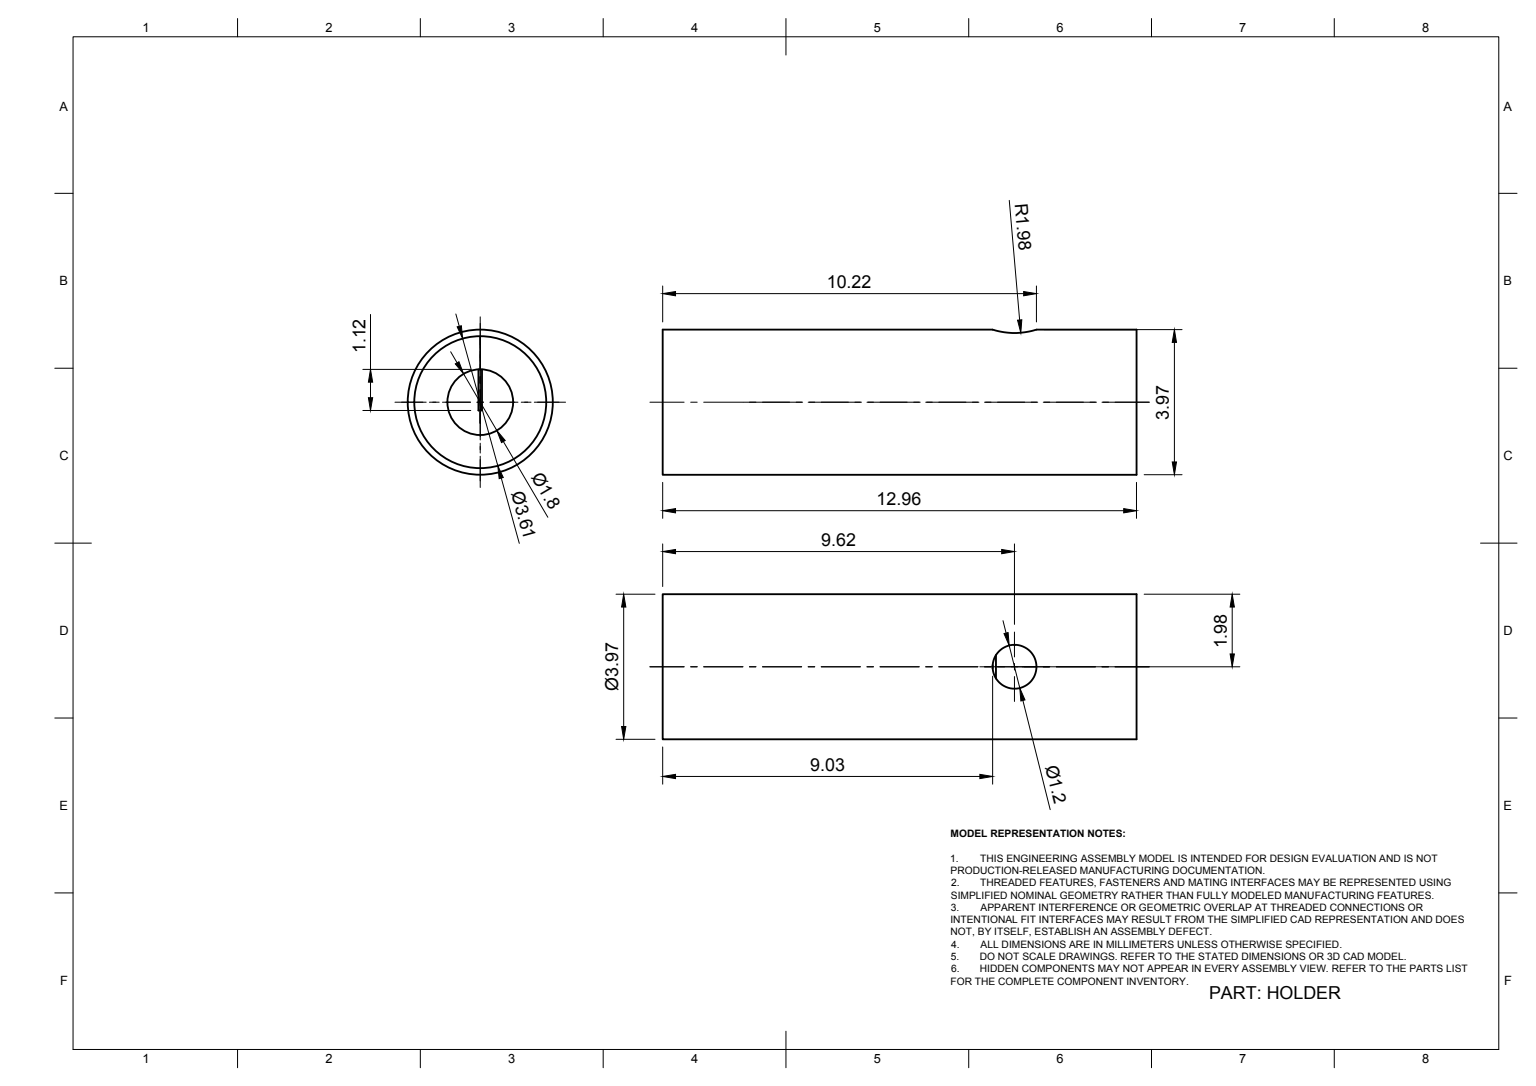
ISO-10303-21;
HEADER;
/* Generated by software containing ST-Developer
 * from STEP Tools, Inc. (www.steptools.com) 
 */

FILE_DESCRIPTION(
/* description */ (''),
/* implementation_level */ '2;1');

FILE_NAME(
/* name */ 'Holder.step',
/* time_stamp */ '2026-10-05T00:51:14-07:00',
/* author */ (''),
/* organization */ (''),
/* preprocessor_version */ 'ST-DEVELOPER v20.2',
/* originating_system */ 'Autodesk Translation Framework v15.15.0.0',
/* authorisation */ '');

FILE_SCHEMA (('AUTOMOTIVE_DESIGN { 1 0 10303 214 3 1 1 }'));
ENDSEC;

DATA;
#10=MECHANICAL_DESIGN_GEOMETRIC_PRESENTATION_REPRESENTATION('',(#388),#4613);
#48=CONICAL_SURFACE('',#1711,1.35128847266969,0.789744339373133);
#67=FACE_BOUND('',#517,.T.);
#68=FACE_BOUND('',#522,.T.);
#69=FACE_BOUND('',#525,.T.);
#70=FACE_BOUND('',#528,.T.);
#91=PLANE('',#1698);
#92=PLANE('',#1702);
#93=PLANE('',#1706);
#94=PLANE('',#1707);
#95=PLANE('',#1715);
#96=PLANE('',#1719);
#97=PLANE('',#1723);
#98=PLANE('',#1727);
#132=B_SPLINE_CURVE_WITH_KNOTS('',3,(#2423,#2424,#2425,#2426,#2427,#2428),
 .UNSPECIFIED.,.F.,.F.,(4,2,4),(0.0611341523507192,0.0707646671678304,0.089396591469994),
 .UNSPECIFIED.);
#133=B_SPLINE_CURVE_WITH_KNOTS('',3,(#2432,#2433,#2434,#2435,#2436,#2437,
#2438,#2439,#2440,#2441,#2442,#2443,#2444,#2445,#2446,#2447,#2448),
 .UNSPECIFIED.,.F.,.F.,(4,2,2,2,3,2,2,4),(-0.0922607888499982,-0.0692273118115021,
-0.0461938347730059,-0.023096917386503,0.,0.023096917386503,0.0461938347730059,
0.0596041129805193),.UNSPECIFIED.);
#134=B_SPLINE_CURVE_WITH_KNOTS('',3,(#2452,#2453,#2454,#2455,#2456,#2457,
#2458,#2459,#2460,#2461),.UNSPECIFIED.,.F.,.F.,(4,2,2,2,4),(0.,0.0227593204764388,
0.0455186409528775,0.0682709506447675,0.0910232603366575),.UNSPECIFIED.);
#135=B_SPLINE_CURVE_WITH_KNOTS('',3,(#2463,#2464,#2465,#2466,#2467,#2468,
#2469,#2470,#2471,#2472),.UNSPECIFIED.,.F.,.F.,(4,2,2,2,4),(0.273069781009973,
0.295822090701863,0.318574400393753,0.341333720870191,0.36409304134663),
 .UNSPECIFIED.);
#136=B_SPLINE_CURVE_WITH_KNOTS('',3,(#2473,#2474,#2475,#2476,#2477,#2478,
#2479,#2480,#2481,#2482,#2483,#2484,#2485,#2486,#2487,#2488,#2489,#2490),
 .UNSPECIFIED.,.F.,.F.,(4,2,2,2,2,2,2,2,4),(0.0910232603366575,0.113775570028548,
0.136527879720438,0.159287200196876,0.182046520673315,0.204805841149754,
0.227565161626193,0.250317471318083,0.273069781009973),.UNSPECIFIED.);
#137=B_SPLINE_CURVE_WITH_KNOTS('',3,(#2492,#2493,#2494,#2495,#2496,#2497,
#2498,#2499,#2500,#2501,#2502,#2503,#2504,#2505,#2506,#2507),
 .UNSPECIFIED.,.F.,.F.,(4,2,2,2,2,2,2,4),(-0.244125690634136,-0.230715412473002,
-0.207618495086499,-0.184521577699996,-0.161424660313493,-0.13832774292699,
-0.115294265888494,-0.0922607888499982),.UNSPECIFIED.);
#138=B_SPLINE_CURVE_WITH_KNOTS('',3,(#2510,#2511,#2512,#2513,#2514,#2515),
 .UNSPECIFIED.,.F.,.F.,(4,2,4),(0.0989596757247573,0.117591600026921,0.127222114844032),
 .UNSPECIFIED.);
#165=LINE('',#2417,#248);
#166=LINE('',#2421,#249);
#167=LINE('',#2430,#250);
#168=LINE('',#2450,#251);
#169=LINE('',#2509,#252);
#170=LINE('',#2517,#253);
#171=LINE('',#2521,#254);
#172=LINE('',#2534,#255);
#173=LINE('',#2537,#256);
#174=LINE('',#2542,#257);
#175=LINE('',#2549,#258);
#176=LINE('',#2550,#259);
#177=LINE('',#2557,#260);
#178=LINE('',#2564,#261);
#248=VECTOR('',#1914,10.);
#249=VECTOR('',#1917,10.);
#250=VECTOR('',#1918,10.);
#251=VECTOR('',#1919,0.600000000000001);
#252=VECTOR('',#1920,10.);
#253=VECTOR('',#1923,10.);
#254=VECTOR('',#1928,1.19802042656629);
#255=VECTOR('',#1949,0.898903149093028);
#256=VECTOR('',#1952,1.35128847266969);
#257=VECTOR('',#1959,1.80367379624636);
#258=VECTOR('',#1968,1.9840612380693);
#259=VECTOR('',#1969,1.9840612380693);
#260=VECTOR('',#1978,1.49577760563294);
#261=VECTOR('',#1987,1.24385197034191);
#331=CYLINDRICAL_SURFACE('',#1696,0.600000000000001);
#332=CYLINDRICAL_SURFACE('',#1699,1.19802042656629);
#333=CYLINDRICAL_SURFACE('',#1704,0.898903149093028);
#334=CYLINDRICAL_SURFACE('',#1709,0.898903149093028);
#335=CYLINDRICAL_SURFACE('',#1713,1.80367379624636);
#336=CYLINDRICAL_SURFACE('',#1717,1.9840612380693);
#337=CYLINDRICAL_SURFACE('',#1721,1.49577760563294);
#338=CYLINDRICAL_SURFACE('',#1725,1.24385197034191);
#372=SHAPE_REPRESENTATION_RELATIONSHIP('SRR','None',#4646,#380);
#380=ADVANCED_BREP_SHAPE_REPRESENTATION('',(#396),#4606);
#388=STYLED_ITEM('',(#4695),#396);
#396=MANIFOLD_SOLID_BREP('Body1',#1595);
#404=FACE_OUTER_BOUND('',#510,.T.);
#405=FACE_OUTER_BOUND('',#511,.T.);
#406=FACE_OUTER_BOUND('',#512,.T.);
#407=FACE_OUTER_BOUND('',#513,.T.);
#408=FACE_OUTER_BOUND('',#514,.T.);
#409=FACE_OUTER_BOUND('',#515,.T.);
#410=FACE_OUTER_BOUND('',#516,.T.);
#411=FACE_OUTER_BOUND('',#518,.T.);
#412=FACE_OUTER_BOUND('',#519,.T.);
#413=FACE_OUTER_BOUND('',#520,.T.);
#414=FACE_OUTER_BOUND('',#521,.T.);
#415=FACE_OUTER_BOUND('',#523,.T.);
#416=FACE_OUTER_BOUND('',#524,.T.);
#417=FACE_OUTER_BOUND('',#526,.T.);
#418=FACE_OUTER_BOUND('',#527,.T.);
#419=FACE_OUTER_BOUND('',#529,.T.);
#420=FACE_OUTER_BOUND('',#530,.T.);
#510=EDGE_LOOP('',(#1073,#1074,#1075,#1076,#1077,#1078,#1079,#1080,#1081,
#1082,#1083,#1084,#1085,#1086));
#511=EDGE_LOOP('',(#1087,#1088));
#512=EDGE_LOOP('',(#1089,#1090,#1091,#1092,#1093,#1094));
#513=EDGE_LOOP('',(#1095,#1096,#1097,#1098));
#514=EDGE_LOOP('',(#1099,#1100,#1101,#1102));
#515=EDGE_LOOP('',(#1103,#1104,#1105,#1106));
#516=EDGE_LOOP('',(#1107));
#517=EDGE_LOOP('',(#1108));
#518=EDGE_LOOP('',(#1109,#1110,#1111,#1112));
#519=EDGE_LOOP('',(#1113,#1114,#1115,#1116));
#520=EDGE_LOOP('',(#1117,#1118,#1119,#1120));
#521=EDGE_LOOP('',(#1121));
#522=EDGE_LOOP('',(#1122));
#523=EDGE_LOOP('',(#1123,#1124,#1125,#1126,#1127,#1128,#1129,#1130,#1131));
#524=EDGE_LOOP('',(#1132));
#525=EDGE_LOOP('',(#1133));
#526=EDGE_LOOP('',(#1134,#1135,#1136,#1137));
#527=EDGE_LOOP('',(#1138));
#528=EDGE_LOOP('',(#1139));
#529=EDGE_LOOP('',(#1140,#1141,#1142,#1143));
#530=EDGE_LOOP('',(#1144));
#640=CIRCLE('',#1697,0.600000000000001);
#641=CIRCLE('',#1700,1.19802042656629);
#642=CIRCLE('',#1701,1.19802042656629);
#643=CIRCLE('',#1703,0.898903149093028);
#644=CIRCLE('',#1705,0.898903149093028);
#645=CIRCLE('',#1708,0.898903149093028);
#646=CIRCLE('',#1710,0.898903149093028);
#647=CIRCLE('',#1712,1.80367379624636);
#648=CIRCLE('',#1714,1.80367379624636);
#649=CIRCLE('',#1716,1.9840612380693);
#650=CIRCLE('',#1718,1.9840612380693);
#651=CIRCLE('',#1720,1.49577760563294);
#652=CIRCLE('',#1722,1.49577760563294);
#653=CIRCLE('',#1724,1.24385197034191);
#654=CIRCLE('',#1726,1.24385197034191);
#733=VERTEX_POINT('',#2415);
#734=VERTEX_POINT('',#2416);
#735=VERTEX_POINT('',#2418);
#736=VERTEX_POINT('',#2420);
#737=VERTEX_POINT('',#2422);
#738=VERTEX_POINT('',#2429);
#739=VERTEX_POINT('',#2431);
#740=VERTEX_POINT('',#2449);
#741=VERTEX_POINT('',#2451);
#742=VERTEX_POINT('',#2462);
#743=VERTEX_POINT('',#2491);
#744=VERTEX_POINT('',#2508);
#745=VERTEX_POINT('',#2519);
#746=VERTEX_POINT('',#2529);
#747=VERTEX_POINT('',#2532);
#748=VERTEX_POINT('',#2536);
#749=VERTEX_POINT('',#2540);
#750=VERTEX_POINT('',#2544);
#751=VERTEX_POINT('',#2547);
#752=VERTEX_POINT('',#2552);
#753=VERTEX_POINT('',#2555);
#754=VERTEX_POINT('',#2559);
#755=VERTEX_POINT('',#2562);
#864=EDGE_CURVE('',#733,#734,#165,.T.);
#865=EDGE_CURVE('',#733,#735,#640,.T.);
#866=EDGE_CURVE('',#736,#735,#166,.T.);
#867=EDGE_CURVE('',#737,#736,#132,.T.);
#868=EDGE_CURVE('',#738,#737,#167,.T.);
#869=EDGE_CURVE('',#739,#738,#133,.T.);
#870=EDGE_CURVE('',#739,#740,#168,.T.);
#871=EDGE_CURVE('',#741,#740,#134,.T.);
#872=EDGE_CURVE('',#742,#741,#135,.T.);
#873=EDGE_CURVE('',#740,#742,#136,.T.);
#874=EDGE_CURVE('',#743,#739,#137,.T.);
#875=EDGE_CURVE('',#744,#743,#169,.T.);
#876=EDGE_CURVE('',#734,#744,#138,.T.);
#877=EDGE_CURVE('',#735,#733,#170,.T.);
#878=EDGE_CURVE('',#745,#745,#641,.T.);
#879=EDGE_CURVE('',#745,#739,#171,.T.);
#880=EDGE_CURVE('',#738,#743,#642,.T.);
#881=EDGE_CURVE('',#736,#734,#643,.T.);
#882=EDGE_CURVE('',#737,#744,#644,.T.);
#883=EDGE_CURVE('',#746,#746,#645,.T.);
#884=EDGE_CURVE('',#747,#747,#646,.T.);
#885=EDGE_CURVE('',#747,#746,#172,.T.);
#886=EDGE_CURVE('',#747,#748,#173,.T.);
#887=EDGE_CURVE('',#748,#748,#647,.T.);
#888=EDGE_CURVE('',#749,#749,#648,.T.);
#889=EDGE_CURVE('',#749,#748,#174,.T.);
#890=EDGE_CURVE('',#750,#750,#649,.T.);
#891=EDGE_CURVE('',#751,#751,#650,.T.);
#892=EDGE_CURVE('',#751,#742,#175,.T.);
#893=EDGE_CURVE('',#740,#750,#176,.T.);
#894=EDGE_CURVE('',#752,#752,#651,.T.);
#895=EDGE_CURVE('',#753,#753,#652,.T.);
#896=EDGE_CURVE('',#753,#752,#177,.T.);
#897=EDGE_CURVE('',#754,#754,#653,.T.);
#898=EDGE_CURVE('',#755,#755,#654,.T.);
#899=EDGE_CURVE('',#755,#754,#178,.T.);
#1073=ORIENTED_EDGE('',*,*,#864,.F.);
#1074=ORIENTED_EDGE('',*,*,#865,.T.);
#1075=ORIENTED_EDGE('',*,*,#866,.F.);
#1076=ORIENTED_EDGE('',*,*,#867,.F.);
#1077=ORIENTED_EDGE('',*,*,#868,.F.);
#1078=ORIENTED_EDGE('',*,*,#869,.F.);
#1079=ORIENTED_EDGE('',*,*,#870,.T.);
#1080=ORIENTED_EDGE('',*,*,#871,.F.);
#1081=ORIENTED_EDGE('',*,*,#872,.F.);
#1082=ORIENTED_EDGE('',*,*,#873,.F.);
#1083=ORIENTED_EDGE('',*,*,#870,.F.);
#1084=ORIENTED_EDGE('',*,*,#874,.F.);
#1085=ORIENTED_EDGE('',*,*,#875,.F.);
#1086=ORIENTED_EDGE('',*,*,#876,.F.);
#1087=ORIENTED_EDGE('',*,*,#877,.F.);
#1088=ORIENTED_EDGE('',*,*,#865,.F.);
#1089=ORIENTED_EDGE('',*,*,#878,.F.);
#1090=ORIENTED_EDGE('',*,*,#879,.T.);
#1091=ORIENTED_EDGE('',*,*,#869,.T.);
#1092=ORIENTED_EDGE('',*,*,#880,.T.);
#1093=ORIENTED_EDGE('',*,*,#874,.T.);
#1094=ORIENTED_EDGE('',*,*,#879,.F.);
#1095=ORIENTED_EDGE('',*,*,#864,.T.);
#1096=ORIENTED_EDGE('',*,*,#881,.F.);
#1097=ORIENTED_EDGE('',*,*,#866,.T.);
#1098=ORIENTED_EDGE('',*,*,#877,.T.);
#1099=ORIENTED_EDGE('',*,*,#876,.T.);
#1100=ORIENTED_EDGE('',*,*,#882,.F.);
#1101=ORIENTED_EDGE('',*,*,#867,.T.);
#1102=ORIENTED_EDGE('',*,*,#881,.T.);
#1103=ORIENTED_EDGE('',*,*,#875,.T.);
#1104=ORIENTED_EDGE('',*,*,#880,.F.);
#1105=ORIENTED_EDGE('',*,*,#868,.T.);
#1106=ORIENTED_EDGE('',*,*,#882,.T.);
#1107=ORIENTED_EDGE('',*,*,#878,.T.);
#1108=ORIENTED_EDGE('',*,*,#883,.F.);
#1109=ORIENTED_EDGE('',*,*,#884,.F.);
#1110=ORIENTED_EDGE('',*,*,#885,.T.);
#1111=ORIENTED_EDGE('',*,*,#883,.T.);
#1112=ORIENTED_EDGE('',*,*,#885,.F.);
#1113=ORIENTED_EDGE('',*,*,#884,.T.);
#1114=ORIENTED_EDGE('',*,*,#886,.T.);
#1115=ORIENTED_EDGE('',*,*,#887,.F.);
#1116=ORIENTED_EDGE('',*,*,#886,.F.);
#1117=ORIENTED_EDGE('',*,*,#888,.F.);
#1118=ORIENTED_EDGE('',*,*,#889,.T.);
#1119=ORIENTED_EDGE('',*,*,#887,.T.);
#1120=ORIENTED_EDGE('',*,*,#889,.F.);
#1121=ORIENTED_EDGE('',*,*,#890,.F.);
#1122=ORIENTED_EDGE('',*,*,#888,.T.);
#1123=ORIENTED_EDGE('',*,*,#891,.F.);
#1124=ORIENTED_EDGE('',*,*,#892,.T.);
#1125=ORIENTED_EDGE('',*,*,#872,.T.);
#1126=ORIENTED_EDGE('',*,*,#871,.T.);
#1127=ORIENTED_EDGE('',*,*,#893,.T.);
#1128=ORIENTED_EDGE('',*,*,#890,.T.);
#1129=ORIENTED_EDGE('',*,*,#893,.F.);
#1130=ORIENTED_EDGE('',*,*,#873,.T.);
#1131=ORIENTED_EDGE('',*,*,#892,.F.);
#1132=ORIENTED_EDGE('',*,*,#891,.T.);
#1133=ORIENTED_EDGE('',*,*,#894,.F.);
#1134=ORIENTED_EDGE('',*,*,#895,.F.);
#1135=ORIENTED_EDGE('',*,*,#896,.T.);
#1136=ORIENTED_EDGE('',*,*,#894,.T.);
#1137=ORIENTED_EDGE('',*,*,#896,.F.);
#1138=ORIENTED_EDGE('',*,*,#895,.T.);
#1139=ORIENTED_EDGE('',*,*,#897,.F.);
#1140=ORIENTED_EDGE('',*,*,#898,.F.);
#1141=ORIENTED_EDGE('',*,*,#899,.T.);
#1142=ORIENTED_EDGE('',*,*,#897,.T.);
#1143=ORIENTED_EDGE('',*,*,#899,.F.);
#1144=ORIENTED_EDGE('',*,*,#898,.T.);
#1489=ADVANCED_FACE('',(#404),#331,.F.);
#1490=ADVANCED_FACE('',(#405),#91,.T.);
#1491=ADVANCED_FACE('',(#406),#332,.F.);
#1492=ADVANCED_FACE('',(#407),#92,.T.);
#1493=ADVANCED_FACE('',(#408),#333,.F.);
#1494=ADVANCED_FACE('',(#409),#93,.T.);
#1495=ADVANCED_FACE('',(#410,#67),#94,.T.);
#1496=ADVANCED_FACE('',(#411),#334,.F.);
#1497=ADVANCED_FACE('',(#412),#48,.F.);
#1498=ADVANCED_FACE('',(#413),#335,.F.);
#1499=ADVANCED_FACE('',(#414,#68),#95,.T.);
#1500=ADVANCED_FACE('',(#415),#336,.T.);
#1501=ADVANCED_FACE('',(#416,#69),#96,.T.);
#1502=ADVANCED_FACE('',(#417),#337,.F.);
#1503=ADVANCED_FACE('',(#418,#70),#97,.T.);
#1504=ADVANCED_FACE('',(#419),#338,.F.);
#1505=ADVANCED_FACE('',(#420),#98,.T.);
#1595=CLOSED_SHELL('',(#1489,#1490,#1491,#1492,#1493,#1494,#1495,#1496,
#1497,#1498,#1499,#1500,#1501,#1502,#1503,#1504,#1505));
#1695=AXIS2_PLACEMENT_3D('',#2413,#1910,#1911);
#1696=AXIS2_PLACEMENT_3D('',#2414,#1912,#1913);
#1697=AXIS2_PLACEMENT_3D('',#2419,#1915,#1916);
#1698=AXIS2_PLACEMENT_3D('',#2516,#1921,#1922);
#1699=AXIS2_PLACEMENT_3D('',#2518,#1924,#1925);
#1700=AXIS2_PLACEMENT_3D('',#2520,#1926,#1927);
#1701=AXIS2_PLACEMENT_3D('',#2522,#1929,#1930);
#1702=AXIS2_PLACEMENT_3D('',#2523,#1931,#1932);
#1703=AXIS2_PLACEMENT_3D('',#2524,#1933,#1934);
#1704=AXIS2_PLACEMENT_3D('',#2525,#1935,#1936);
#1705=AXIS2_PLACEMENT_3D('',#2526,#1937,#1938);
#1706=AXIS2_PLACEMENT_3D('',#2527,#1939,#1940);
#1707=AXIS2_PLACEMENT_3D('',#2528,#1941,#1942);
#1708=AXIS2_PLACEMENT_3D('',#2530,#1943,#1944);
#1709=AXIS2_PLACEMENT_3D('',#2531,#1945,#1946);
#1710=AXIS2_PLACEMENT_3D('',#2533,#1947,#1948);
#1711=AXIS2_PLACEMENT_3D('',#2535,#1950,#1951);
#1712=AXIS2_PLACEMENT_3D('',#2538,#1953,#1954);
#1713=AXIS2_PLACEMENT_3D('',#2539,#1955,#1956);
#1714=AXIS2_PLACEMENT_3D('',#2541,#1957,#1958);
#1715=AXIS2_PLACEMENT_3D('',#2543,#1960,#1961);
#1716=AXIS2_PLACEMENT_3D('',#2545,#1962,#1963);
#1717=AXIS2_PLACEMENT_3D('',#2546,#1964,#1965);
#1718=AXIS2_PLACEMENT_3D('',#2548,#1966,#1967);
#1719=AXIS2_PLACEMENT_3D('',#2551,#1970,#1971);
#1720=AXIS2_PLACEMENT_3D('',#2553,#1972,#1973);
#1721=AXIS2_PLACEMENT_3D('',#2554,#1974,#1975);
#1722=AXIS2_PLACEMENT_3D('',#2556,#1976,#1977);
#1723=AXIS2_PLACEMENT_3D('',#2558,#1979,#1980);
#1724=AXIS2_PLACEMENT_3D('',#2560,#1981,#1982);
#1725=AXIS2_PLACEMENT_3D('',#2561,#1983,#1984);
#1726=AXIS2_PLACEMENT_3D('',#2563,#1985,#1986);
#1727=AXIS2_PLACEMENT_3D('',#2565,#1988,#1989);
#1910=DIRECTION('axis',(0.,0.,1.));
#1911=DIRECTION('refdir',(1.,0.,0.));
#1912=DIRECTION('center_axis',(0.,0.,1.));
#1913=DIRECTION('ref_axis',(1.,0.,0.));
#1914=DIRECTION('',(0.,0.,1.));
#1915=DIRECTION('center_axis',(0.,0.,-1.));
#1916=DIRECTION('ref_axis',(1.,0.,0.));
#1917=DIRECTION('',(0.,0.,-1.));
#1918=DIRECTION('',(0.,0.,-1.));
#1919=DIRECTION('',(0.,0.,1.));
#1920=DIRECTION('',(0.,0.,1.));
#1921=DIRECTION('center_axis',(0.,0.,1.));
#1922=DIRECTION('ref_axis',(1.,0.,0.));
#1923=DIRECTION('',(0.,1.,0.));
#1924=DIRECTION('center_axis',(1.,0.,0.));
#1925=DIRECTION('ref_axis',(0.,0.,-1.));
#1926=DIRECTION('center_axis',(1.,0.,0.));
#1927=DIRECTION('ref_axis',(0.,0.,-1.));
#1928=DIRECTION('',(1.,0.,0.));
#1929=DIRECTION('center_axis',(1.,0.,0.));
#1930=DIRECTION('ref_axis',(0.,0.,-1.));
#1931=DIRECTION('center_axis',(-1.,0.,0.));
#1932=DIRECTION('ref_axis',(0.,0.,1.));
#1933=DIRECTION('center_axis',(1.,0.,0.));
#1934=DIRECTION('ref_axis',(0.,0.,-1.));
#1935=DIRECTION('center_axis',(1.,0.,0.));
#1936=DIRECTION('ref_axis',(0.,0.,-1.));
#1937=DIRECTION('center_axis',(1.,0.,0.));
#1938=DIRECTION('ref_axis',(0.,0.,-1.));
#1939=DIRECTION('center_axis',(-1.,0.,0.));
#1940=DIRECTION('ref_axis',(0.,0.,1.));
#1941=DIRECTION('center_axis',(1.,0.,0.));
#1942=DIRECTION('ref_axis',(0.,0.,-1.));
#1943=DIRECTION('center_axis',(1.,0.,0.));
#1944=DIRECTION('ref_axis',(0.,0.,-1.));
#1945=DIRECTION('center_axis',(1.,0.,0.));
#1946=DIRECTION('ref_axis',(0.,0.,-1.));
#1947=DIRECTION('center_axis',(1.,0.,0.));
#1948=DIRECTION('ref_axis',(0.,0.,-1.));
#1949=DIRECTION('',(1.,0.,0.));
#1950=DIRECTION('center_axis',(-1.,0.,0.));
#1951=DIRECTION('ref_axis',(0.,0.,-1.));
#1952=DIRECTION('',(-0.704026902010687,8.69711463179084E-17,0.710173303669769));
#1953=DIRECTION('center_axis',(1.,0.,0.));
#1954=DIRECTION('ref_axis',(0.,0.,-1.));
#1955=DIRECTION('center_axis',(1.,0.,0.));
#1956=DIRECTION('ref_axis',(0.,0.,-1.));
#1957=DIRECTION('center_axis',(1.,0.,0.));
#1958=DIRECTION('ref_axis',(0.,0.,-1.));
#1959=DIRECTION('',(1.,0.,0.));
#1960=DIRECTION('center_axis',(-1.,0.,0.));
#1961=DIRECTION('ref_axis',(0.,0.,1.));
#1962=DIRECTION('center_axis',(1.,0.,0.));
#1963=DIRECTION('ref_axis',(0.,0.,-1.));
#1964=DIRECTION('center_axis',(1.,0.,0.));
#1965=DIRECTION('ref_axis',(0.,0.,-1.));
#1966=DIRECTION('center_axis',(1.,0.,0.));
#1967=DIRECTION('ref_axis',(0.,0.,-1.));
#1968=DIRECTION('',(-1.,0.,0.));
#1969=DIRECTION('',(-1.,0.,0.));
#1970=DIRECTION('center_axis',(1.,0.,0.));
#1971=DIRECTION('ref_axis',(0.,0.,-1.));
#1972=DIRECTION('center_axis',(1.,0.,0.));
#1973=DIRECTION('ref_axis',(0.,0.,-1.));
#1974=DIRECTION('center_axis',(1.,0.,0.));
#1975=DIRECTION('ref_axis',(0.,0.,-1.));
#1976=DIRECTION('center_axis',(1.,0.,0.));
#1977=DIRECTION('ref_axis',(0.,0.,-1.));
#1978=DIRECTION('',(1.,0.,0.));
#1979=DIRECTION('center_axis',(1.,0.,0.));
#1980=DIRECTION('ref_axis',(0.,0.,-1.));
#1981=DIRECTION('center_axis',(1.,0.,0.));
#1982=DIRECTION('ref_axis',(0.,0.,-1.));
#1983=DIRECTION('center_axis',(1.,0.,0.));
#1984=DIRECTION('ref_axis',(0.,0.,-1.));
#1985=DIRECTION('center_axis',(1.,0.,0.));
#1986=DIRECTION('ref_axis',(0.,0.,-1.));
#1987=DIRECTION('',(1.,0.,0.));
#1988=DIRECTION('center_axis',(1.,0.,0.));
#1989=DIRECTION('ref_axis',(0.,0.,-1.));
#2413=CARTESIAN_POINT('',(0.,0.,0.));
#2414=CARTESIAN_POINT('Origin',(-25.2637346688979,0.,1.77272245287895));
#2415=CARTESIAN_POINT('',(-24.6656713617233,0.0481692911654238,-0.227277547121048));
#2416=CARTESIAN_POINT('',(-24.6656713617233,0.0481692911654247,0.897611603555783));
#2417=CARTESIAN_POINT('',(-24.6656713617233,0.0481692911654238,1.77272245287895));
#2418=CARTESIAN_POINT('',(-24.6656713617233,-0.0481692911654238,-0.227277547121048));
#2419=CARTESIAN_POINT('Origin',(-25.2637346688979,0.,-0.227277547121048));
#2420=CARTESIAN_POINT('',(-24.6656713617233,-0.0481692911654247,0.897611603555783));
#2421=CARTESIAN_POINT('',(-24.6656713617233,-0.0481692911654238,1.77272245287895));
#2422=CARTESIAN_POINT('',(-24.7560377201621,-0.319755857247933,0.840108959126733));
#2423=CARTESIAN_POINT('Ctrl Pts',(-24.7560377201621,-0.319755857247933,
0.840108959126733));
#2424=CARTESIAN_POINT('Ctrl Pts',(-24.7389020605853,-0.292548467970954,
0.850464427887334));
#2425=CARTESIAN_POINT('Ctrl Pts',(-24.7237010096035,-0.263521886093109,
0.859980342899897));
#2426=CARTESIAN_POINT('Ctrl Pts',(-24.686207592206,-0.174658036922562,0.883855860882441));
#2427=CARTESIAN_POINT('Ctrl Pts',(-24.6707368006861,-0.111061086022905,
0.894236587940559));
#2428=CARTESIAN_POINT('Ctrl Pts',(-24.6656713617233,-0.0481692911654243,
0.897611603555783));
#2429=CARTESIAN_POINT('',(-24.7560377201621,-0.319755857247933,1.15456014751321));
#2430=CARTESIAN_POINT('',(-24.7560377201621,-0.319755857247933,1.77272245287895));
#2431=CARTESIAN_POINT('',(-25.8637346688979,-6.49286604591722E-17,1.19802042656629));
#2432=CARTESIAN_POINT('Ctrl Pts',(-25.8637346688979,-5.63785129692462E-17,
1.19802042656629));
#2433=CARTESIAN_POINT('Ctrl Pts',(-25.8637346688979,-0.0767782567949871,
1.19802042656629));
#2434=CARTESIAN_POINT('Ctrl Pts',(-25.8481109979872,-0.157774416814917,
1.18996152111882));
#2435=CARTESIAN_POINT('Ctrl Pts',(-25.7864300204004,-0.30525073804353,1.16091479971318));
#2436=CARTESIAN_POINT('Ctrl Pts',(-25.7404416616373,-0.371821144684504,
1.14023972009026));
#2437=CARTESIAN_POINT('Ctrl Pts',(-25.6354113717621,-0.476851434559632,
1.10046700926426));
#2438=CARTESIAN_POINT('Ctrl Pts',(-25.5688895915929,-0.522733853172129,
1.07852127007884));
#2439=CARTESIAN_POINT('Ctrl Pts',(-25.4216260093517,-0.584328998785629,
1.04643134391016));
#2440=CARTESIAN_POINT('Ctrl Pts',(-25.3407243935196,-0.600000000000001,
1.03694404018253));
#2441=CARTESIAN_POINT('Ctrl Pts',(-25.2637346688979,-0.600000000000001,
1.03694404018253));
#2442=CARTESIAN_POINT('Ctrl Pts',(-25.1867449442762,-0.600000000000001,
1.03694404018253));
#2443=CARTESIAN_POINT('Ctrl Pts',(-25.1058433284441,-0.584328998785631,
1.04643134391016));
#2444=CARTESIAN_POINT('Ctrl Pts',(-24.9585797462029,-0.522733853172133,
1.07852127007884));
#2445=CARTESIAN_POINT('Ctrl Pts',(-24.8920579660337,-0.476851434559632,
1.10046700926426));
#2446=CARTESIAN_POINT('Ctrl Pts',(-24.8089379020593,-0.393731370585291,
1.13194278898667));
#2447=CARTESIAN_POINT('Ctrl Pts',(-24.7804480917521,-0.358513774867966,
1.14382612798167));
#2448=CARTESIAN_POINT('Ctrl Pts',(-24.7560377201621,-0.319755857247933,
1.15456014751321));
#2449=CARTESIAN_POINT('',(-25.8637346688979,-7.34788079488413E-17,1.9840612380693));
#2450=CARTESIAN_POINT('',(-25.8637346688979,-7.34788079488413E-17,1.77272245287895));
#2451=CARTESIAN_POINT('',(-25.2637346688979,-0.600000000000001,1.89116339759659));
#2452=CARTESIAN_POINT('Ctrl Pts',(-25.2637346688979,-0.600000000000001,
1.89116339759659));
#2453=CARTESIAN_POINT('Ctrl Pts',(-25.339599070486,-0.600000000000001,1.89116339759659));
#2454=CARTESIAN_POINT('Ctrl Pts',(-25.4201684023226,-0.584740786326485,
1.89620635355867));
#2455=CARTESIAN_POINT('Ctrl Pts',(-25.5678391532475,-0.523367759786817,
1.91405498074209));
#2456=CARTESIAN_POINT('Ctrl Pts',(-25.6349858006078,-0.477277005713967,
1.926564479109));
#2457=CARTESIAN_POINT('Ctrl Pts',(-25.7409953444987,-0.371267461823086,
1.94976990694802));
#2458=CARTESIAN_POINT('Ctrl Pts',(-25.7870987390016,-0.3041141877551,1.9620248365967));
#2459=CARTESIAN_POINT('Ctrl Pts',(-25.8484811044704,-0.156419315054409,
1.97928267214026));
#2460=CARTESIAN_POINT('Ctrl Pts',(-25.8637346688979,-0.0758410323063,1.9840612380693));
#2461=CARTESIAN_POINT('Ctrl Pts',(-25.8637346688979,8.23993651088983E-17,
1.9840612380693));
#2462=CARTESIAN_POINT('',(-24.6637346688979,-1.12815094845811E-16,1.9840612380693));
#2463=CARTESIAN_POINT('Ctrl Pts',(-24.6637346688979,1.73472347600281E-17,
1.9840612380693));
#2464=CARTESIAN_POINT('Ctrl Pts',(-24.6637346688979,-0.0758410323063,1.9840612380693));
#2465=CARTESIAN_POINT('Ctrl Pts',(-24.6789882333254,-0.156419315054409,
1.97928267214026));
#2466=CARTESIAN_POINT('Ctrl Pts',(-24.7403705987942,-0.304114187755101,
1.9620248365967));
#2467=CARTESIAN_POINT('Ctrl Pts',(-24.7864739932971,-0.371267461823086,
1.94976990694802));
#2468=CARTESIAN_POINT('Ctrl Pts',(-24.892483537188,-0.477277005713967,1.926564479109));
#2469=CARTESIAN_POINT('Ctrl Pts',(-24.9596301845483,-0.523367759786817,
1.91405498074209));
#2470=CARTESIAN_POINT('Ctrl Pts',(-25.1073009354732,-0.584740786326485,
1.89620635355867));
#2471=CARTESIAN_POINT('Ctrl Pts',(-25.1878702673098,-0.600000000000001,
1.89116339759659));
#2472=CARTESIAN_POINT('Ctrl Pts',(-25.2637346688979,-0.600000000000001,
1.89116339759659));
#2473=CARTESIAN_POINT('Ctrl Pts',(-25.8637346688979,8.23993651088983E-17,
1.9840612380693));
#2474=CARTESIAN_POINT('Ctrl Pts',(-25.8637346688979,0.0758410323063001,
1.9840612380693));
#2475=CARTESIAN_POINT('Ctrl Pts',(-25.8484811044704,0.156419315054409,1.97928267214026));
#2476=CARTESIAN_POINT('Ctrl Pts',(-25.7870987390016,0.304114187755101,1.9620248365967));
#2477=CARTESIAN_POINT('Ctrl Pts',(-25.7409953444987,0.371267461823086,1.94976990694802));
#2478=CARTESIAN_POINT('Ctrl Pts',(-25.6349858006078,0.477277005713967,1.926564479109));
#2479=CARTESIAN_POINT('Ctrl Pts',(-25.5678391532475,0.523367759786817,1.91405498074209));
#2480=CARTESIAN_POINT('Ctrl Pts',(-25.4201684023226,0.584740786326485,1.89620635355867));
#2481=CARTESIAN_POINT('Ctrl Pts',(-25.339599070486,0.600000000000001,1.89116339759659));
#2482=CARTESIAN_POINT('Ctrl Pts',(-25.1878702673098,0.600000000000001,1.89116339759659));
#2483=CARTESIAN_POINT('Ctrl Pts',(-25.1073009354732,0.584740786326485,1.89620635355867));
#2484=CARTESIAN_POINT('Ctrl Pts',(-24.9596301845483,0.523367759786817,1.91405498074209));
#2485=CARTESIAN_POINT('Ctrl Pts',(-24.892483537188,0.477277005713967,1.926564479109));
#2486=CARTESIAN_POINT('Ctrl Pts',(-24.7864739932971,0.371267461823086,1.94976990694802));
#2487=CARTESIAN_POINT('Ctrl Pts',(-24.7403705987942,0.304114187755098,1.9620248365967));
#2488=CARTESIAN_POINT('Ctrl Pts',(-24.6789882333254,0.156419315054404,1.97928267214026));
#2489=CARTESIAN_POINT('Ctrl Pts',(-24.6637346688979,0.0758410323063001,
1.9840612380693));
#2490=CARTESIAN_POINT('Ctrl Pts',(-24.6637346688979,1.73472347597681E-17,
1.9840612380693));
#2491=CARTESIAN_POINT('',(-24.7560377201621,0.319755857247933,1.15456014751321));
#2492=CARTESIAN_POINT('Ctrl Pts',(-24.7560377201621,0.319755857247933,1.15456014751321));
#2493=CARTESIAN_POINT('Ctrl Pts',(-24.7804480917171,0.358513774812489,1.14382612799704));
#2494=CARTESIAN_POINT('Ctrl Pts',(-24.8089379021649,0.393731370690889,1.13194278894668));
#2495=CARTESIAN_POINT('Ctrl Pts',(-24.8920579660337,0.476851434559632,1.10046700926426));
#2496=CARTESIAN_POINT('Ctrl Pts',(-24.9585797462029,0.522733853172133,1.07852127007884));
#2497=CARTESIAN_POINT('Ctrl Pts',(-25.1058433284441,0.584328998785631,1.04643134391016));
#2498=CARTESIAN_POINT('Ctrl Pts',(-25.1867449442762,0.600000000000001,1.03694404018253));
#2499=CARTESIAN_POINT('Ctrl Pts',(-25.3407243935196,0.600000000000001,1.03694404018253));
#2500=CARTESIAN_POINT('Ctrl Pts',(-25.4216260093517,0.584328998785631,1.04643134391016));
#2501=CARTESIAN_POINT('Ctrl Pts',(-25.5688895915929,0.522733853172133,1.07852127007884));
#2502=CARTESIAN_POINT('Ctrl Pts',(-25.6354113717621,0.476851434559632,1.10046700926426));
#2503=CARTESIAN_POINT('Ctrl Pts',(-25.7404416616373,0.371821144684504,1.14023972009026));
#2504=CARTESIAN_POINT('Ctrl Pts',(-25.7864300204004,0.305250738043532,1.16091479971318));
#2505=CARTESIAN_POINT('Ctrl Pts',(-25.8481109979872,0.157774416814918,1.18996152111882));
#2506=CARTESIAN_POINT('Ctrl Pts',(-25.8637346688979,0.076778256794987,1.19802042656629));
#2507=CARTESIAN_POINT('Ctrl Pts',(-25.8637346688979,-5.63785129695031E-17,
1.19802042656629));
#2508=CARTESIAN_POINT('',(-24.7560377201621,0.319755857247933,0.840108959126733));
#2509=CARTESIAN_POINT('',(-24.7560377201621,0.319755857247933,1.77272245287895));
#2510=CARTESIAN_POINT('Ctrl Pts',(-24.6656713617233,0.0481692911654243,
0.897611603555783));
#2511=CARTESIAN_POINT('Ctrl Pts',(-24.6707368006861,0.111061086022906,0.894236587940559));
#2512=CARTESIAN_POINT('Ctrl Pts',(-24.686207592206,0.174658036922562,0.883855860882441));
#2513=CARTESIAN_POINT('Ctrl Pts',(-24.7237010096035,0.263521886093109,0.859980342899897));
#2514=CARTESIAN_POINT('Ctrl Pts',(-24.7389020605853,0.292548467970953,0.850464427887335));
#2515=CARTESIAN_POINT('Ctrl Pts',(-24.7560377201621,0.319755857247933,0.840108959126733));
#2516=CARTESIAN_POINT('Origin',(-25.2637346688979,0.,-0.227277547121048));
#2517=CARTESIAN_POINT('',(-24.6656713617233,0.,-0.227277547121048));
#2518=CARTESIAN_POINT('Origin',(-25.5549741096415,0.,0.));
#2519=CARTESIAN_POINT('',(-26.3539104991209,-1.46715188070755E-16,1.19802042656629));
#2520=CARTESIAN_POINT('Origin',(-26.3539104991209,0.,0.));
#2521=CARTESIAN_POINT('',(-25.5549741096415,-1.46715188070755E-16,1.19802042656629));
#2522=CARTESIAN_POINT('Origin',(-24.7560377201621,0.,0.));
#2523=CARTESIAN_POINT('Origin',(-24.6656713617233,0.,-0.898903149093028));
#2524=CARTESIAN_POINT('Origin',(-24.6656713617233,0.,0.));
#2525=CARTESIAN_POINT('Origin',(-24.7108545409427,0.,0.));
#2526=CARTESIAN_POINT('Origin',(-24.7560377201621,0.,0.));
#2527=CARTESIAN_POINT('Origin',(-24.7560377201621,0.,-1.19802042656629));
#2528=CARTESIAN_POINT('Origin',(-26.3539104991209,0.,-0.898903149093028));
#2529=CARTESIAN_POINT('',(-26.3539104991209,-1.10083886428025E-16,0.898903149093028));
#2530=CARTESIAN_POINT('Origin',(-26.3539104991209,0.,0.));
#2531=CARTESIAN_POINT('Origin',(-26.5296283843145,0.,0.));
#2532=CARTESIAN_POINT('',(-26.7053462695082,-1.10083886428025E-16,0.898903149093028));
#2533=CARTESIAN_POINT('Origin',(-26.7053462695082,0.,0.));
#2534=CARTESIAN_POINT('',(-26.5296283843145,-1.10083886428025E-16,0.898903149093028));
#2535=CARTESIAN_POINT('Origin',(-27.1538162925674,0.,0.));
#2536=CARTESIAN_POINT('',(-27.6022863156265,-2.20886334127906E-16,1.80367379624636));
#2537=CARTESIAN_POINT('',(-27.1538162925674,1.65485110277965E-16,1.35128847266969));
#2538=CARTESIAN_POINT('Origin',(-27.6022863156265,0.,0.));
#2539=CARTESIAN_POINT('Origin',(-28.1016442624067,0.,0.));
#2540=CARTESIAN_POINT('',(-28.6010022091869,-2.20886334127906E-16,1.80367379624636));
#2541=CARTESIAN_POINT('Origin',(-28.6010022091869,0.,0.));
#2542=CARTESIAN_POINT('',(-28.1016442624067,-2.20886334127906E-16,1.80367379624636));
#2543=CARTESIAN_POINT('Origin',(-28.6010022091869,0.,-1.9840612380693));
#2544=CARTESIAN_POINT('',(-28.6010022091869,-2.4297742445139E-16,1.9840612380693));
#2545=CARTESIAN_POINT('Origin',(-28.6010022091869,0.,0.));
#2546=CARTESIAN_POINT('Origin',(-22.120782962919,0.,0.));
#2547=CARTESIAN_POINT('',(-15.6405637166511,-2.4297742445139E-16,1.9840612380693));
#2548=CARTESIAN_POINT('Origin',(-15.6405637166511,0.,0.));
#2549=CARTESIAN_POINT('',(-22.120782962919,-2.4297742445139E-16,1.9840612380693));
#2550=CARTESIAN_POINT('',(-22.120782962919,-2.4297742445139E-16,1.9840612380693));
#2551=CARTESIAN_POINT('Origin',(-15.6405637166511,0.,-1.49577760563294));
#2552=CARTESIAN_POINT('',(-15.6405637166511,-1.83179925697468E-16,1.49577760563294));
#2553=CARTESIAN_POINT('Origin',(-15.6405637166511,0.,0.));
#2554=CARTESIAN_POINT('Origin',(-19.5773288456352,0.,0.));
#2555=CARTESIAN_POINT('',(-23.5140939746193,-1.83179925697468E-16,1.49577760563294));
#2556=CARTESIAN_POINT('Origin',(-23.5140939746193,0.,0.));
#2557=CARTESIAN_POINT('',(-19.5773288456352,-1.83179925697467E-16,1.49577760563294));
#2558=CARTESIAN_POINT('Origin',(-23.5140939746193,0.,-1.24385197034191));
#2559=CARTESIAN_POINT('',(-23.5140939746193,-1.52327933409234E-16,1.24385197034191));
#2560=CARTESIAN_POINT('Origin',(-23.5140939746193,0.,0.));
#2561=CARTESIAN_POINT('Origin',(-23.8926057114429,0.,0.));
#2562=CARTESIAN_POINT('',(-24.2711174482666,-1.52327933409234E-16,1.24385197034191));
#2563=CARTESIAN_POINT('Origin',(-24.2711174482666,0.,0.));
#2564=CARTESIAN_POINT('',(-23.8926057114429,-1.52327933409235E-16,1.24385197034191));
#2565=CARTESIAN_POINT('Origin',(-24.2711174482666,0.,0.));
#4596=UNCERTAINTY_MEASURE_WITH_UNIT(LENGTH_MEASURE(0.01),#4614,
'DISTANCE_ACCURACY_VALUE',
'Maximum model space distance between geometric entities at asserted c
onnectivities');
#4603=UNCERTAINTY_MEASURE_WITH_UNIT(LENGTH_MEASURE(0.01),#4614,
'DISTANCE_ACCURACY_VALUE',
'Maximum model space distance between geometric entities at asserted c
onnectivities');
#4606=(
GEOMETRIC_REPRESENTATION_CONTEXT(3)
GLOBAL_UNCERTAINTY_ASSIGNED_CONTEXT((#4596))
GLOBAL_UNIT_ASSIGNED_CONTEXT((#4614,#4616,#4617))
REPRESENTATION_CONTEXT('','3D')
);
#4613=(
GEOMETRIC_REPRESENTATION_CONTEXT(3)
GLOBAL_UNCERTAINTY_ASSIGNED_CONTEXT((#4603))
GLOBAL_UNIT_ASSIGNED_CONTEXT((#4614,#4616,#4617))
REPRESENTATION_CONTEXT('','3D')
);
#4614=(
LENGTH_UNIT()
NAMED_UNIT(*)
SI_UNIT(.MILLI.,.METRE.)
);
#4616=(
NAMED_UNIT(*)
PLANE_ANGLE_UNIT()
SI_UNIT($,.RADIAN.)
);
#4617=(
NAMED_UNIT(*)
SI_UNIT($,.STERADIAN.)
SOLID_ANGLE_UNIT()
);
#4620=SHAPE_DEFINITION_REPRESENTATION(#4629,#4646);
#4629=PRODUCT_DEFINITION_SHAPE('',$,#4656);
#4646=SHAPE_REPRESENTATION('',(#1695),#4606);
#4653=PRODUCT_DEFINITION_CONTEXT('part definition',#4682,'design');
#4656=PRODUCT_DEFINITION('Holder','Holder',#4665,#4653);
#4665=PRODUCT_DEFINITION_FORMATION('',$,#4686);
#4682=APPLICATION_CONTEXT(
'Core Data for Automotive Mechanical Design Process');
#4683=PRODUCT_CONTEXT('part definition',#4682,'mechanical');
#4686=PRODUCT('Holder','Holder',$,(#4683));
#4695=PRESENTATION_STYLE_ASSIGNMENT((#4700));
#4700=SURFACE_STYLE_USAGE(.BOTH.,#4705);
#4705=SURFACE_SIDE_STYLE('',(#4710));
#4710=SURFACE_STYLE_FILL_AREA(#4715);
#4715=FILL_AREA_STYLE('Opaque(255,255,255)',(#4720));
#4720=FILL_AREA_STYLE_COLOUR('Opaque(255,255,255)',#4725);
#4725=COLOUR_RGB('Opaque(255,255,255)', 0.66274510, 0.83137255, 0.94901961);
ENDSEC;
END-ISO-10303-21;
